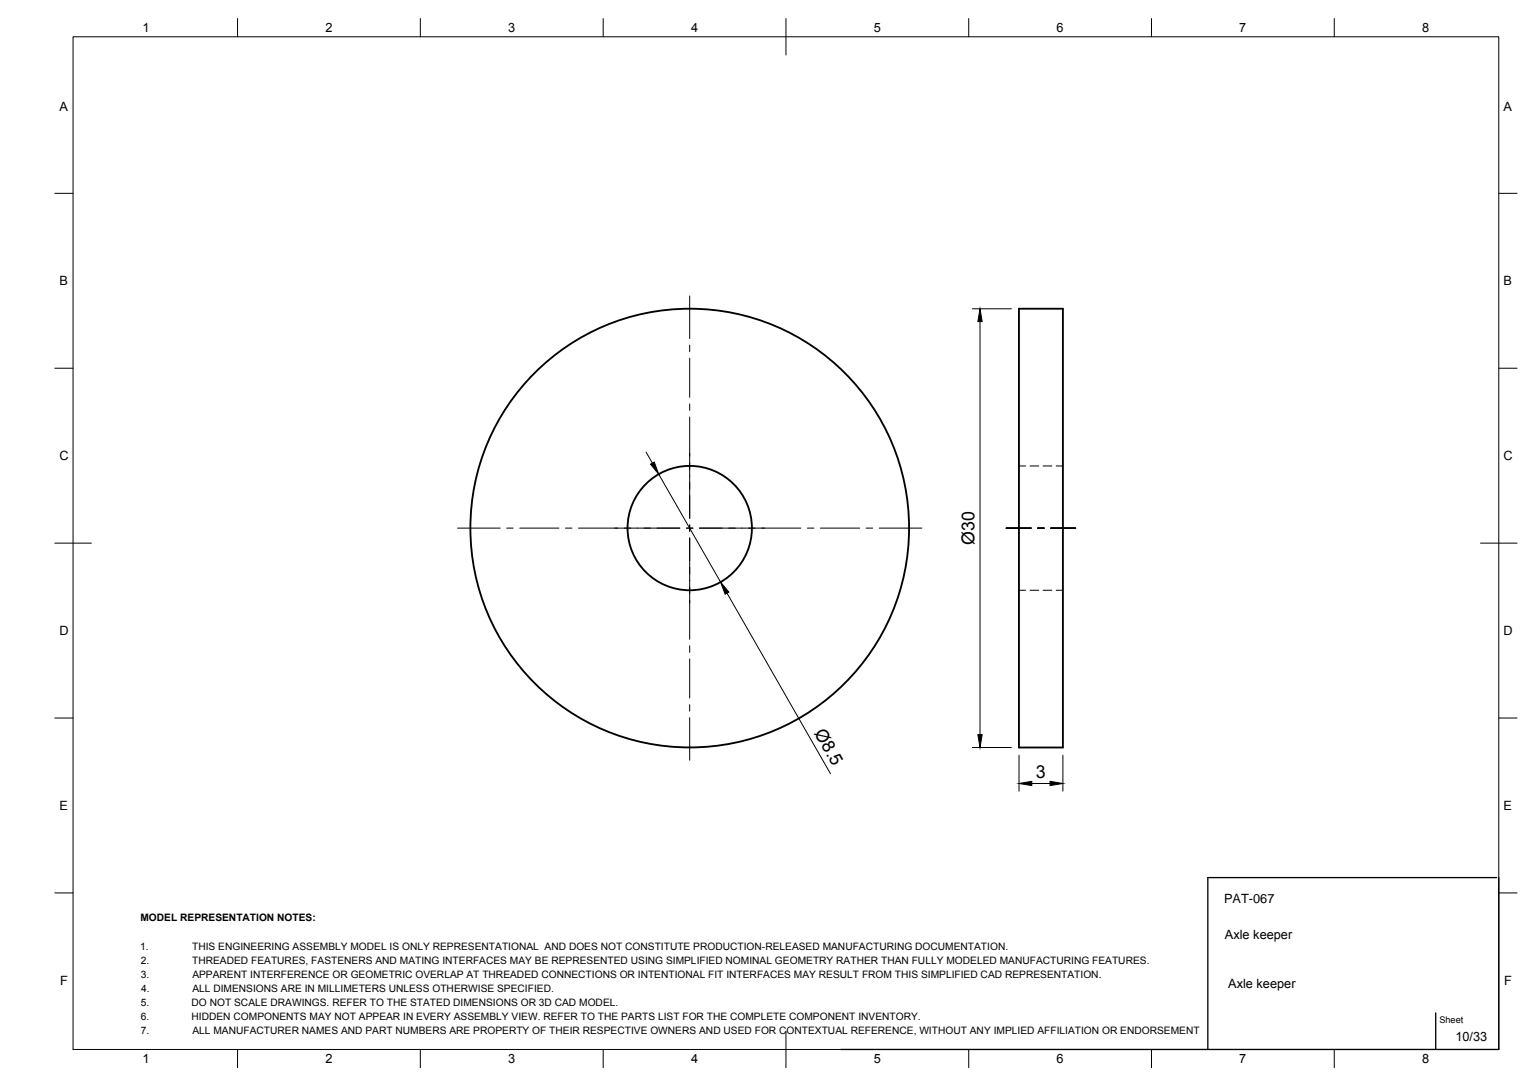
ISO-10303-21;
HEADER;
/* Generated by software containing ST-Developer
 * from STEP Tools, Inc. (www.steptools.com) 
 */

FILE_DESCRIPTION(
/* description */ ('Lifting hook block with sheave'),
/* implementation_level */ '2;1');

FILE_NAME(
/* name */ 'Axle keeper.step',
/* time_stamp */ '2026-10-28T03:23:54-07:00',
/* author */ (''),
/* organization */ (''),
/* preprocessor_version */ 'ST-DEVELOPER v20.2',
/* originating_system */ 'Autodesk Translation Framework v15.17.0.0',
/* authorisation */ '');

FILE_SCHEMA (('AUTOMOTIVE_DESIGN { 1 0 10303 214 3 1 1 }'));
ENDSEC;

DATA;
#10=MECHANICAL_DESIGN_GEOMETRIC_PRESENTATION_REPRESENTATION('',(#356),#9391);
#296=SHAPE_REPRESENTATION_RELATIONSHIP('SRR','None',#9527,#326);
#326=ADVANCED_BREP_SHAPE_REPRESENTATION('',(#394),#9362);
#356=STYLED_ITEM('',(#9759),#394);
#394=MANIFOLD_SOLID_BREP('Body1',#4892);
#526=LINE('',#7949,#814);
#527=LINE('',#7955,#815);
#814=VECTOR('',#6359,0.425);
#815=VECTOR('',#6366,1.5);
#1034=CYLINDRICAL_SURFACE('',#5421,0.425);
#1035=CYLINDRICAL_SURFACE('',#5424,1.5);
#1145=FACE_BOUND('',#1622,.T.);
#1146=FACE_BOUND('',#1624,.T.);
#1292=FACE_OUTER_BOUND('',#1619,.T.);
#1293=FACE_OUTER_BOUND('',#1620,.T.);
#1294=FACE_OUTER_BOUND('',#1621,.T.);
#1295=FACE_OUTER_BOUND('',#1623,.T.);
#1619=EDGE_LOOP('',(#3602,#3603,#3604,#3605));
#1620=EDGE_LOOP('',(#3606,#3607,#3608,#3609));
#1621=EDGE_LOOP('',(#3610));
#1622=EDGE_LOOP('',(#3611));
#1623=EDGE_LOOP('',(#3612));
#1624=EDGE_LOOP('',(#3613));
#1999=CIRCLE('',#5422,0.425);
#2000=CIRCLE('',#5423,0.425);
#2001=CIRCLE('',#5425,1.5);
#2002=CIRCLE('',#5426,1.5);
#2332=VERTEX_POINT('',#7946);
#2333=VERTEX_POINT('',#7948);
#2334=VERTEX_POINT('',#7952);
#2335=VERTEX_POINT('',#7954);
#2805=EDGE_CURVE('',#2332,#2332,#1999,.T.);
#2806=EDGE_CURVE('',#2332,#2333,#526,.T.);
#2807=EDGE_CURVE('',#2333,#2333,#2000,.T.);
#2808=EDGE_CURVE('',#2334,#2334,#2001,.T.);
#2809=EDGE_CURVE('',#2334,#2335,#527,.T.);
#2810=EDGE_CURVE('',#2335,#2335,#2002,.T.);
#3602=ORIENTED_EDGE('',*,*,#2805,.F.);
#3603=ORIENTED_EDGE('',*,*,#2806,.T.);
#3604=ORIENTED_EDGE('',*,*,#2807,.T.);
#3605=ORIENTED_EDGE('',*,*,#2806,.F.);
#3606=ORIENTED_EDGE('',*,*,#2808,.F.);
#3607=ORIENTED_EDGE('',*,*,#2809,.T.);
#3608=ORIENTED_EDGE('',*,*,#2810,.T.);
#3609=ORIENTED_EDGE('',*,*,#2809,.F.);
#3610=ORIENTED_EDGE('',*,*,#2808,.T.);
#3611=ORIENTED_EDGE('',*,*,#2805,.T.);
#3612=ORIENTED_EDGE('',*,*,#2810,.F.);
#3613=ORIENTED_EDGE('',*,*,#2807,.F.);
#4488=PLANE('',#5427);
#4489=PLANE('',#5428);
#4668=ADVANCED_FACE('',(#1292),#1034,.F.);
#4669=ADVANCED_FACE('',(#1293),#1035,.T.);
#4670=ADVANCED_FACE('',(#1294,#1145),#4488,.T.);
#4671=ADVANCED_FACE('',(#1295,#1146),#4489,.F.);
#4892=CLOSED_SHELL('',(#4668,#4669,#4670,#4671));
#5420=AXIS2_PLACEMENT_3D('',#7944,#6353,#6354);
#5421=AXIS2_PLACEMENT_3D('',#7945,#6355,#6356);
#5422=AXIS2_PLACEMENT_3D('',#7947,#6357,#6358);
#5423=AXIS2_PLACEMENT_3D('',#7950,#6360,#6361);
#5424=AXIS2_PLACEMENT_3D('',#7951,#6362,#6363);
#5425=AXIS2_PLACEMENT_3D('',#7953,#6364,#6365);
#5426=AXIS2_PLACEMENT_3D('',#7956,#6367,#6368);
#5427=AXIS2_PLACEMENT_3D('',#7957,#6369,#6370);
#5428=AXIS2_PLACEMENT_3D('',#7958,#6371,#6372);
#6353=DIRECTION('axis',(0.,0.,1.));
#6354=DIRECTION('refdir',(1.,0.,0.));
#6355=DIRECTION('center_axis',(0.,1.,0.));
#6356=DIRECTION('ref_axis',(1.,0.,0.));
#6357=DIRECTION('center_axis',(0.,-1.,0.));
#6358=DIRECTION('ref_axis',(1.,0.,0.));
#6359=DIRECTION('',(0.,-1.,0.));
#6360=DIRECTION('center_axis',(0.,-1.,0.));
#6361=DIRECTION('ref_axis',(1.,0.,0.));
#6362=DIRECTION('center_axis',(0.,1.,0.));
#6363=DIRECTION('ref_axis',(1.,0.,0.));
#6364=DIRECTION('center_axis',(0.,1.,0.));
#6365=DIRECTION('ref_axis',(1.,0.,0.));
#6366=DIRECTION('',(0.,-1.,0.));
#6367=DIRECTION('center_axis',(0.,1.,0.));
#6368=DIRECTION('ref_axis',(1.,0.,0.));
#6369=DIRECTION('center_axis',(0.,1.,0.));
#6370=DIRECTION('ref_axis',(1.,0.,0.));
#6371=DIRECTION('center_axis',(0.,1.,0.));
#6372=DIRECTION('ref_axis',(1.,0.,0.));
#7944=CARTESIAN_POINT('',(0.,0.,0.));
#7945=CARTESIAN_POINT('Origin',(0.,3.1,12.));
#7946=CARTESIAN_POINT('',(-0.425,3.4,12.));
#7947=CARTESIAN_POINT('Origin',(0.,3.4,12.));
#7948=CARTESIAN_POINT('',(-0.425,3.1,12.));
#7949=CARTESIAN_POINT('',(-0.425,3.1,12.));
#7950=CARTESIAN_POINT('Origin',(0.,3.1,12.));
#7951=CARTESIAN_POINT('Origin',(0.,3.1,12.));
#7952=CARTESIAN_POINT('',(-1.5,3.4,12.));
#7953=CARTESIAN_POINT('Origin',(0.,3.4,12.));
#7954=CARTESIAN_POINT('',(-1.5,3.1,12.));
#7955=CARTESIAN_POINT('',(-1.5,3.1,12.));
#7956=CARTESIAN_POINT('Origin',(0.,3.1,12.));
#7957=CARTESIAN_POINT('Origin',(0.,3.4,12.));
#7958=CARTESIAN_POINT('Origin',(0.,3.1,12.));
#9325=UNCERTAINTY_MEASURE_WITH_UNIT(LENGTH_MEASURE(0.001),#9392,
'DISTANCE_ACCURACY_VALUE',
'Maximum model space distance between geometric entities at asserted c
onnectivities');
#9354=UNCERTAINTY_MEASURE_WITH_UNIT(LENGTH_MEASURE(0.001),#9392,
'DISTANCE_ACCURACY_VALUE',
'Maximum model space distance between geometric entities at asserted c
onnectivities');
#9362=(
GEOMETRIC_REPRESENTATION_CONTEXT(3)
GLOBAL_UNCERTAINTY_ASSIGNED_CONTEXT((#9325))
GLOBAL_UNIT_ASSIGNED_CONTEXT((#9392,#9394,#9395))
REPRESENTATION_CONTEXT('','3D')
);
#9391=(
GEOMETRIC_REPRESENTATION_CONTEXT(3)
GLOBAL_UNCERTAINTY_ASSIGNED_CONTEXT((#9354))
GLOBAL_UNIT_ASSIGNED_CONTEXT((#9392,#9394,#9395))
REPRESENTATION_CONTEXT('','3D')
);
#9392=(
LENGTH_UNIT()
NAMED_UNIT(*)
SI_UNIT(.CENTI.,.METRE.)
);
#9394=(
NAMED_UNIT(*)
PLANE_ANGLE_UNIT()
SI_UNIT($,.RADIAN.)
);
#9395=(
NAMED_UNIT(*)
SI_UNIT($,.STERADIAN.)
SOLID_ANGLE_UNIT()
);
#9403=SHAPE_DEFINITION_REPRESENTATION(#9439,#9527);
#9439=PRODUCT_DEFINITION_SHAPE('',$,#9564);
#9527=SHAPE_REPRESENTATION('',(#5420),#9362);
#9556=PRODUCT_DEFINITION_CONTEXT('part definition',#9666,'design');
#9564=PRODUCT_DEFINITION('Axle keeper','Axle keeper',#9600,#9556);
#9600=PRODUCT_DEFINITION_FORMATION('',$,#9675);
#9666=APPLICATION_CONTEXT(
'Core Data for Automotive Mechanical Design Process');
#9667=PRODUCT_CONTEXT('part definition',#9666,'mechanical');
#9675=PRODUCT('Axle keeper','Axle keeper','Axle keeper',(#9667));
#9753=COLOUR_RGB('Grey',0.48,0.52,0.57);
#9754=FILL_AREA_STYLE_COLOUR('',#9753);
#9755=FILL_AREA_STYLE('',(#9754));
#9756=SURFACE_STYLE_FILL_AREA(#9755);
#9757=SURFACE_SIDE_STYLE('',(#9756));
#9758=SURFACE_STYLE_USAGE(.BOTH.,#9757);
#9759=PRESENTATION_STYLE_ASSIGNMENT((#9758));
ENDSEC;
END-ISO-10303-21;
